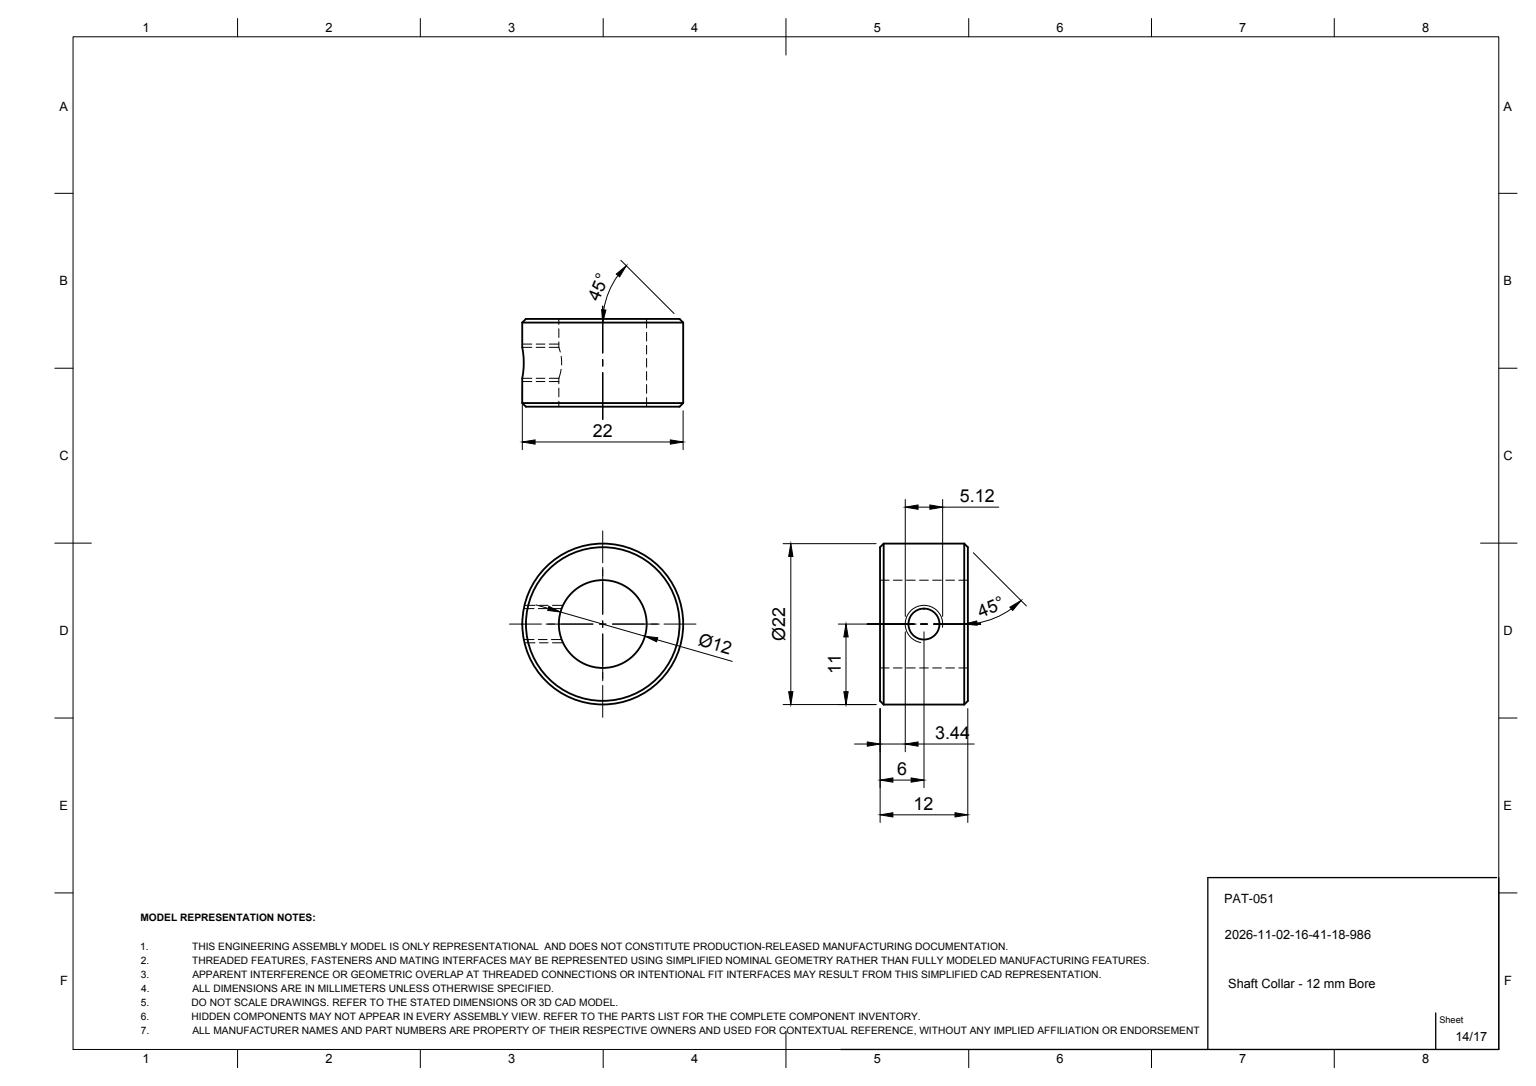
ISO-10303-21;
HEADER;
/* Generated by software containing ST-Developer
 * from STEP Tools, Inc. (www.steptools.com) 
 */

FILE_DESCRIPTION(
/* description */ ('Hand-crank flanged shaft unit'),
/* implementation_level */ '2;1');

FILE_NAME(
/* name */ 'Shaft Collar - 12 mm Bore.step',
/* time_stamp */ '2026-10-27T18:35:45-07:00',
/* author */ (''),
/* organization */ (''),
/* preprocessor_version */ 'ST-DEVELOPER v20.2',
/* originating_system */ 'Autodesk Translation Framework v15.17.0.0',
/* authorisation */ '');

FILE_SCHEMA (('AUTOMOTIVE_DESIGN { 1 0 10303 214 3 1 1 }'));
ENDSEC;

DATA;
#10=MECHANICAL_DESIGN_GEOMETRIC_PRESENTATION_REPRESENTATION('',(#298),#6805);
#24=CONICAL_SURFACE('',#3900,1.075,0.785398163397448);
#25=CONICAL_SURFACE('',#3904,1.075,0.785398163397449);
#235=B_SPLINE_CURVE_WITH_KNOTS('',3,(#6600,#6601,#6602,#6603,#6604,#6605,
#6606,#6607,#6608,#6609,#6610,#6611,#6612,#6613,#6614,#6615,#6616,#6617,
#6618,#6619,#6620,#6621,#6622,#6623,#6624,#6625,#6626,#6627,#6628,#6629,
#6630,#6631,#6632,#6633),.UNSPECIFIED.,.T.,.F.,(4,2,2,2,2,2,2,2,2,2,2,2,
2,2,2,2,4),(0.,0.0805240527913139,0.161048105582628,0.241524630728584,0.322001155874541,
0.402477681020498,0.482954206166455,0.563478258957768,0.644002311749082,
0.724526364540396,0.80505041733171,0.885526942477667,0.966003467623624,
1.04647999276958,1.12695651791554,1.20748057070685,1.28800462349816),
 .UNSPECIFIED.);
#236=B_SPLINE_CURVE_WITH_KNOTS('',3,(#6636,#6637,#6638,#6639,#6640,#6641,
#6642,#6643,#6644,#6645,#6646,#6647,#6648,#6649,#6650,#6651,#6652,#6653,
#6654,#6655,#6656,#6657,#6658,#6659,#6660,#6661,#6662,#6663,#6664,#6665,
#6666,#6667,#6668,#6669),.UNSPECIFIED.,.T.,.F.,(4,2,2,2,2,2,2,2,2,2,2,2,
2,2,2,2,4),(0.,0.0799614062161292,0.159922812432258,0.239880387792505,0.319837963152752,
0.399795538512999,0.479753113873245,0.559714520089374,0.639675926305503,
0.719637332521632,0.799598738737761,0.879556314098008,0.959513889458255,
1.0394714648185,1.11942904017875,1.19939044639488,1.27935185261101),
 .UNSPECIFIED.);
#257=SHAPE_REPRESENTATION_RELATIONSHIP('SRR','None',#6920,#277);
#277=ADVANCED_BREP_SHAPE_REPRESENTATION('',(#318),#6803);
#298=STYLED_ITEM('',(#7091),#318);
#318=MANIFOLD_SOLID_BREP('Body1',#3340);
#405=FACE_BOUND('',#959,.T.);
#406=FACE_BOUND('',#962,.T.);
#407=FACE_BOUND('',#965,.T.);
#408=FACE_BOUND('',#967,.T.);
#504=PLANE('',#3897);
#505=PLANE('',#3906);
#684=FACE_OUTER_BOUND('',#957,.T.);
#685=FACE_OUTER_BOUND('',#958,.T.);
#686=FACE_OUTER_BOUND('',#960,.T.);
#687=FACE_OUTER_BOUND('',#961,.T.);
#688=FACE_OUTER_BOUND('',#963,.T.);
#689=FACE_OUTER_BOUND('',#964,.T.);
#690=FACE_OUTER_BOUND('',#966,.T.);
#957=EDGE_LOOP('',(#2991,#2992,#2993,#2994));
#958=EDGE_LOOP('',(#2995));
#959=EDGE_LOOP('',(#2996));
#960=EDGE_LOOP('',(#2997,#2998,#2999,#3000));
#961=EDGE_LOOP('',(#3001,#3002,#3003,#3004));
#962=EDGE_LOOP('',(#3005));
#963=EDGE_LOOP('',(#3006,#3007,#3008,#3009));
#964=EDGE_LOOP('',(#3010));
#965=EDGE_LOOP('',(#3011));
#966=EDGE_LOOP('',(#3012,#3013,#3014,#3015));
#967=EDGE_LOOP('',(#3016));
#1183=LINE('',#6635,#1411);
#1184=LINE('',#6678,#1412);
#1185=LINE('',#6682,#1413);
#1186=LINE('',#6686,#1414);
#1187=LINE('',#6691,#1415);
#1411=VECTOR('',#4828,0.21);
#1412=VECTOR('',#4839,1.075);
#1413=VECTOR('',#4844,1.1);
#1414=VECTOR('',#4849,1.075);
#1415=VECTOR('',#4856,0.6);
#1559=CIRCLE('',#3898,1.05);
#1560=CIRCLE('',#3899,0.6);
#1561=CIRCLE('',#3901,1.1);
#1562=CIRCLE('',#3903,1.1);
#1563=CIRCLE('',#3905,1.05);
#1564=CIRCLE('',#3907,0.6);
#1819=VERTEX_POINT('',#6599);
#1820=VERTEX_POINT('',#6634);
#1821=VERTEX_POINT('',#6671);
#1822=VERTEX_POINT('',#6673);
#1823=VERTEX_POINT('',#6676);
#1824=VERTEX_POINT('',#6680);
#1825=VERTEX_POINT('',#6684);
#1826=VERTEX_POINT('',#6688);
#2213=EDGE_CURVE('',#1819,#1819,#235,.T.);
#2214=EDGE_CURVE('',#1819,#1820,#1183,.T.);
#2215=EDGE_CURVE('',#1820,#1820,#236,.T.);
#2216=EDGE_CURVE('',#1821,#1821,#1559,.T.);
#2217=EDGE_CURVE('',#1822,#1822,#1560,.T.);
#2218=EDGE_CURVE('',#1823,#1823,#1561,.T.);
#2219=EDGE_CURVE('',#1823,#1821,#1184,.T.);
#2220=EDGE_CURVE('',#1824,#1824,#1562,.T.);
#2221=EDGE_CURVE('',#1824,#1823,#1185,.T.);
#2222=EDGE_CURVE('',#1825,#1825,#1563,.T.);
#2223=EDGE_CURVE('',#1825,#1824,#1186,.T.);
#2224=EDGE_CURVE('',#1826,#1826,#1564,.T.);
#2225=EDGE_CURVE('',#1826,#1822,#1187,.T.);
#2991=ORIENTED_EDGE('',*,*,#2213,.F.);
#2992=ORIENTED_EDGE('',*,*,#2214,.T.);
#2993=ORIENTED_EDGE('',*,*,#2215,.F.);
#2994=ORIENTED_EDGE('',*,*,#2214,.F.);
#2995=ORIENTED_EDGE('',*,*,#2216,.F.);
#2996=ORIENTED_EDGE('',*,*,#2217,.T.);
#2997=ORIENTED_EDGE('',*,*,#2218,.F.);
#2998=ORIENTED_EDGE('',*,*,#2219,.T.);
#2999=ORIENTED_EDGE('',*,*,#2216,.T.);
#3000=ORIENTED_EDGE('',*,*,#2219,.F.);
#3001=ORIENTED_EDGE('',*,*,#2220,.F.);
#3002=ORIENTED_EDGE('',*,*,#2221,.T.);
#3003=ORIENTED_EDGE('',*,*,#2218,.T.);
#3004=ORIENTED_EDGE('',*,*,#2221,.F.);
#3005=ORIENTED_EDGE('',*,*,#2215,.T.);
#3006=ORIENTED_EDGE('',*,*,#2222,.F.);
#3007=ORIENTED_EDGE('',*,*,#2223,.T.);
#3008=ORIENTED_EDGE('',*,*,#2220,.T.);
#3009=ORIENTED_EDGE('',*,*,#2223,.F.);
#3010=ORIENTED_EDGE('',*,*,#2222,.T.);
#3011=ORIENTED_EDGE('',*,*,#2224,.F.);
#3012=ORIENTED_EDGE('',*,*,#2224,.T.);
#3013=ORIENTED_EDGE('',*,*,#2225,.T.);
#3014=ORIENTED_EDGE('',*,*,#2217,.F.);
#3015=ORIENTED_EDGE('',*,*,#2225,.F.);
#3016=ORIENTED_EDGE('',*,*,#2213,.T.);
#3128=CYLINDRICAL_SURFACE('',#3896,0.2117);
#3129=CYLINDRICAL_SURFACE('',#3902,1.1);
#3130=CYLINDRICAL_SURFACE('',#3908,0.6);
#3301=ADVANCED_FACE('',(#684),#3128,.F.);
#3302=ADVANCED_FACE('',(#685,#405),#504,.T.);
#3303=ADVANCED_FACE('',(#686),#24,.T.);
#3304=ADVANCED_FACE('',(#687,#406),#3129,.T.);
#3305=ADVANCED_FACE('',(#688),#25,.T.);
#3306=ADVANCED_FACE('',(#689,#407),#505,.T.);
#3307=ADVANCED_FACE('',(#690,#408),#3130,.F.);
#3340=CLOSED_SHELL('',(#3301,#3302,#3303,#3304,#3305,#3306,#3307));
#3895=AXIS2_PLACEMENT_3D('',#6597,#4824,#4825);
#3896=AXIS2_PLACEMENT_3D('',#6598,#4826,#4827);
#3897=AXIS2_PLACEMENT_3D('',#6670,#4829,#4830);
#3898=AXIS2_PLACEMENT_3D('',#6672,#4831,#4832);
#3899=AXIS2_PLACEMENT_3D('',#6674,#4833,#4834);
#3900=AXIS2_PLACEMENT_3D('',#6675,#4835,#4836);
#3901=AXIS2_PLACEMENT_3D('',#6677,#4837,#4838);
#3902=AXIS2_PLACEMENT_3D('',#6679,#4840,#4841);
#3903=AXIS2_PLACEMENT_3D('',#6681,#4842,#4843);
#3904=AXIS2_PLACEMENT_3D('',#6683,#4845,#4846);
#3905=AXIS2_PLACEMENT_3D('',#6685,#4847,#4848);
#3906=AXIS2_PLACEMENT_3D('',#6687,#4850,#4851);
#3907=AXIS2_PLACEMENT_3D('',#6689,#4852,#4853);
#3908=AXIS2_PLACEMENT_3D('',#6690,#4854,#4855);
#4824=DIRECTION('axis',(0.,0.,1.));
#4825=DIRECTION('refdir',(1.,0.,0.));
#4826=DIRECTION('center_axis',(1.,0.,0.));
#4827=DIRECTION('ref_axis',(0.,0.,-1.));
#4828=DIRECTION('',(1.,0.,0.));
#4829=DIRECTION('center_axis',(0.,1.,0.));
#4830=DIRECTION('ref_axis',(0.,0.,1.));
#4831=DIRECTION('center_axis',(0.,-1.,0.));
#4832=DIRECTION('ref_axis',(1.,0.,0.));
#4833=DIRECTION('center_axis',(0.,-1.,0.));
#4834=DIRECTION('ref_axis',(1.,0.,0.));
#4835=DIRECTION('center_axis',(0.,-1.,0.));
#4836=DIRECTION('ref_axis',(1.,0.,0.));
#4837=DIRECTION('center_axis',(0.,-1.,0.));
#4838=DIRECTION('ref_axis',(1.,0.,0.));
#4839=DIRECTION('',(0.707106781186548,0.707106781186547,8.65956056235493E-17));
#4840=DIRECTION('center_axis',(0.,-1.,0.));
#4841=DIRECTION('ref_axis',(1.,0.,0.));
#4842=DIRECTION('center_axis',(0.,-1.,0.));
#4843=DIRECTION('ref_axis',(1.,0.,0.));
#4844=DIRECTION('',(0.,1.,0.));
#4845=DIRECTION('center_axis',(0.,1.,0.));
#4846=DIRECTION('ref_axis',(1.,0.,0.));
#4847=DIRECTION('center_axis',(0.,-1.,0.));
#4848=DIRECTION('ref_axis',(1.,0.,0.));
#4849=DIRECTION('',(-0.707106781186548,0.707106781186547,-8.65956056235494E-17));
#4850=DIRECTION('center_axis',(0.,-1.,0.));
#4851=DIRECTION('ref_axis',(0.,0.,-1.));
#4852=DIRECTION('center_axis',(0.,-1.,0.));
#4853=DIRECTION('ref_axis',(1.,0.,0.));
#4854=DIRECTION('center_axis',(0.,-1.,0.));
#4855=DIRECTION('ref_axis',(1.,0.,0.));
#4856=DIRECTION('',(0.,1.,0.));
#6597=CARTESIAN_POINT('',(0.,0.,0.));
#6598=CARTESIAN_POINT('Origin',(0.5,0.6,0.));
#6599=CARTESIAN_POINT('',(0.561411711669787,0.6,0.2117));
#6600=CARTESIAN_POINT('Ctrl Pts',(0.561411711669787,0.6,0.2117));
#6601=CARTESIAN_POINT('Ctrl Pts',(0.561411711669787,0.573158649069562,0.2117));
#6602=CARTESIAN_POINT('Ctrl Pts',(0.563539297838208,0.544705001203387,0.206288194517509));
#6603=CARTESIAN_POINT('Ctrl Pts',(0.571006257413022,0.492626080621549,0.184616375754799));
#6604=CARTESIAN_POINT('Ctrl Pts',(0.576215579648966,0.468977868958045,0.168366880112429));
#6605=CARTESIAN_POINT('Ctrl Pts',(0.585834170098139,0.431644140867814,0.131033152022198));
#6606=CARTESIAN_POINT('Ctrl Pts',(0.590898115435695,0.41538619377614,0.107380608633747));
#6607=CARTESIAN_POINT('Ctrl Pts',(0.598025669508798,0.393708029332882,0.0552854099234836));
#6608=CARTESIAN_POINT('Ctrl Pts',(0.6,0.3883,0.0268255083819855));
#6609=CARTESIAN_POINT('Ctrl Pts',(0.6,0.3883,-0.0268255083819856));
#6610=CARTESIAN_POINT('Ctrl Pts',(0.598025669508798,0.393708029332882,-0.0552854099234837));
#6611=CARTESIAN_POINT('Ctrl Pts',(0.590898115435695,0.41538619377614,-0.107380608633747));
#6612=CARTESIAN_POINT('Ctrl Pts',(0.585834170098139,0.431644140867814,-0.131033152022198));
#6613=CARTESIAN_POINT('Ctrl Pts',(0.576215579648966,0.468977868958045,-0.168366880112429));
#6614=CARTESIAN_POINT('Ctrl Pts',(0.571006257413022,0.49262608062155,-0.184616375754799));
#6615=CARTESIAN_POINT('Ctrl Pts',(0.563539297838207,0.544705001203387,-0.206288194517509));
#6616=CARTESIAN_POINT('Ctrl Pts',(0.561411711669787,0.573158649069562,-0.2117));
#6617=CARTESIAN_POINT('Ctrl Pts',(0.561411711669787,0.626841350930438,-0.2117));
#6618=CARTESIAN_POINT('Ctrl Pts',(0.563539297838207,0.655294998796613,-0.206288194517509));
#6619=CARTESIAN_POINT('Ctrl Pts',(0.571006257413022,0.70737391937845,-0.184616375754799));
#6620=CARTESIAN_POINT('Ctrl Pts',(0.576215579648966,0.731022131041955,-0.168366880112429));
#6621=CARTESIAN_POINT('Ctrl Pts',(0.585834170098139,0.768355859132186,-0.131033152022198));
#6622=CARTESIAN_POINT('Ctrl Pts',(0.590898115435695,0.78461380622386,-0.107380608633747));
#6623=CARTESIAN_POINT('Ctrl Pts',(0.598025669508798,0.806291970667118,-0.0552854099234837));
#6624=CARTESIAN_POINT('Ctrl Pts',(0.6,0.8117,-0.0268255083819856));
#6625=CARTESIAN_POINT('Ctrl Pts',(0.6,0.8117,0.0268255083819855));
#6626=CARTESIAN_POINT('Ctrl Pts',(0.598025669508798,0.806291970667118,0.0552854099234837));
#6627=CARTESIAN_POINT('Ctrl Pts',(0.590898115435695,0.78461380622386,0.107380608633747));
#6628=CARTESIAN_POINT('Ctrl Pts',(0.585834170098139,0.768355859132186,0.131033152022198));
#6629=CARTESIAN_POINT('Ctrl Pts',(0.576215579648966,0.731022131041955,0.168366880112429));
#6630=CARTESIAN_POINT('Ctrl Pts',(0.571006257413022,0.70737391937845,0.184616375754799));
#6631=CARTESIAN_POINT('Ctrl Pts',(0.563539297838207,0.655294998796613,0.206288194517509));
#6632=CARTESIAN_POINT('Ctrl Pts',(0.561411711669787,0.626841350930438,0.2117));
#6633=CARTESIAN_POINT('Ctrl Pts',(0.561411711669787,0.6,0.2117));
#6634=CARTESIAN_POINT('',(1.07943647798284,0.6,0.2117));
#6635=CARTESIAN_POINT('',(0.5,0.6,0.2117));
#6636=CARTESIAN_POINT('Ctrl Pts',(1.07943647798284,0.6,0.2117));
#6637=CARTESIAN_POINT('Ctrl Pts',(1.07943647798284,0.626653802072043,0.2117));
#6638=CARTESIAN_POINT('Ctrl Pts',(1.08052600621577,0.655037401084091,0.206359582618511));
#6639=CARTESIAN_POINT('Ctrl Pts',(1.08443252298676,0.707175401021015,0.18473448130117));
#6640=CARTESIAN_POINT('Ctrl Pts',(1.08718996287164,0.730935702749545,0.168453308404839));
#6641=CARTESIAN_POINT('Ctrl Pts',(1.09234340045893,0.768452409692904,0.13093660146148));
#6642=CARTESIAN_POINT('Ctrl Pts',(1.09507838311905,0.784734286816328,0.107175917083711));
#6643=CARTESIAN_POINT('Ctrl Pts',(1.09893326276149,0.806359899102434,0.0550365908820453));
#6644=CARTESIAN_POINT('Ctrl Pts',(1.1,0.8117,0.0266525251200821));
#6645=CARTESIAN_POINT('Ctrl Pts',(1.1,0.8117,-0.0266525251200823));
#6646=CARTESIAN_POINT('Ctrl Pts',(1.09893326276149,0.806359899102434,-0.0550365908820454));
#6647=CARTESIAN_POINT('Ctrl Pts',(1.09507838311905,0.784734286816328,-0.107175917083711));
#6648=CARTESIAN_POINT('Ctrl Pts',(1.09234340045893,0.768452409692904,-0.130936601461481));
#6649=CARTESIAN_POINT('Ctrl Pts',(1.08718996287164,0.730935702749545,-0.16845330840484));
#6650=CARTESIAN_POINT('Ctrl Pts',(1.08443252298676,0.707175401021015,-0.18473448130117));
#6651=CARTESIAN_POINT('Ctrl Pts',(1.08052600621577,0.655037401084091,-0.206359582618511));
#6652=CARTESIAN_POINT('Ctrl Pts',(1.07943647798284,0.626653802072043,-0.2117));
#6653=CARTESIAN_POINT('Ctrl Pts',(1.07943647798284,0.573346197927957,-0.2117));
#6654=CARTESIAN_POINT('Ctrl Pts',(1.08052600621577,0.544962598915909,-0.206359582618511));
#6655=CARTESIAN_POINT('Ctrl Pts',(1.08443252298676,0.492824598978985,-0.18473448130117));
#6656=CARTESIAN_POINT('Ctrl Pts',(1.08718996287164,0.469064297250455,-0.168453308404839));
#6657=CARTESIAN_POINT('Ctrl Pts',(1.09234340045893,0.431547590307096,-0.13093660146148));
#6658=CARTESIAN_POINT('Ctrl Pts',(1.09507838311905,0.415265713183672,-0.107175917083711));
#6659=CARTESIAN_POINT('Ctrl Pts',(1.09893326276149,0.393640100897566,-0.0550365908820454));
#6660=CARTESIAN_POINT('Ctrl Pts',(1.1,0.3883,-0.0266525251200822));
#6661=CARTESIAN_POINT('Ctrl Pts',(1.1,0.3883,0.0266525251200823));
#6662=CARTESIAN_POINT('Ctrl Pts',(1.09893326276149,0.393640100897566,0.0550365908820454));
#6663=CARTESIAN_POINT('Ctrl Pts',(1.09507838311905,0.415265713183672,0.107175917083711));
#6664=CARTESIAN_POINT('Ctrl Pts',(1.09234340045893,0.431547590307096,0.13093660146148));
#6665=CARTESIAN_POINT('Ctrl Pts',(1.08718996287164,0.469064297250455,0.16845330840484));
#6666=CARTESIAN_POINT('Ctrl Pts',(1.08443252298676,0.492824598978985,0.18473448130117));
#6667=CARTESIAN_POINT('Ctrl Pts',(1.08052600621577,0.544962598915909,0.206359582618511));
#6668=CARTESIAN_POINT('Ctrl Pts',(1.07943647798284,0.573346197927957,0.2117));
#6669=CARTESIAN_POINT('Ctrl Pts',(1.07943647798284,0.6,0.2117));
#6670=CARTESIAN_POINT('Origin',(1.05,1.2,0.));
#6671=CARTESIAN_POINT('',(-1.05,1.2,-1.28587913910472E-16));
#6672=CARTESIAN_POINT('Origin',(0.,1.2,0.));
#6673=CARTESIAN_POINT('',(-0.6,1.2,-7.34788079488412E-17));
#6674=CARTESIAN_POINT('Origin',(0.,1.2,0.));
#6675=CARTESIAN_POINT('Origin',(0.,1.175,0.));
#6676=CARTESIAN_POINT('',(-1.1,1.15,-1.34711147906209E-16));
#6677=CARTESIAN_POINT('Origin',(0.,1.15,0.));
#6678=CARTESIAN_POINT('',(-1.075,1.175,-1.3164953090834E-16));
#6679=CARTESIAN_POINT('Origin',(0.,0.6,0.));
#6680=CARTESIAN_POINT('',(-1.1,0.05,-1.34711147906209E-16));
#6681=CARTESIAN_POINT('Origin',(0.,0.05,0.));
#6682=CARTESIAN_POINT('',(-1.1,0.6,-1.34711147906209E-16));
#6683=CARTESIAN_POINT('Origin',(0.,0.025,0.));
#6684=CARTESIAN_POINT('',(-1.05,-4.5102810375397E-17,-1.28587913910472E-16));
#6685=CARTESIAN_POINT('Origin',(0.,0.,0.));
#6686=CARTESIAN_POINT('',(-1.075,0.025,-1.3164953090834E-16));
#6687=CARTESIAN_POINT('Origin',(0.6,0.,0.));
#6688=CARTESIAN_POINT('',(-0.6,0.,-7.34788079488412E-17));
#6689=CARTESIAN_POINT('Origin',(0.,0.,0.));
#6690=CARTESIAN_POINT('Origin',(0.,0.6,0.));
#6691=CARTESIAN_POINT('',(-0.6,0.6,-7.34788079488412E-17));
#6778=UNCERTAINTY_MEASURE_WITH_UNIT(LENGTH_MEASURE(0.001),#6806,
'DISTANCE_ACCURACY_VALUE',
'Maximum model space distance between geometric entities at asserted c
onnectivities');
#6780=UNCERTAINTY_MEASURE_WITH_UNIT(LENGTH_MEASURE(0.001),#6806,
'DISTANCE_ACCURACY_VALUE',
'Maximum model space distance between geometric entities at asserted c
onnectivities');
#6803=(
GEOMETRIC_REPRESENTATION_CONTEXT(3)
GLOBAL_UNCERTAINTY_ASSIGNED_CONTEXT((#6778))
GLOBAL_UNIT_ASSIGNED_CONTEXT((#6806,#6808,#6809))
REPRESENTATION_CONTEXT('','3D')
);
#6805=(
GEOMETRIC_REPRESENTATION_CONTEXT(3)
GLOBAL_UNCERTAINTY_ASSIGNED_CONTEXT((#6780))
GLOBAL_UNIT_ASSIGNED_CONTEXT((#6806,#6808,#6809))
REPRESENTATION_CONTEXT('','3D')
);
#6806=(
LENGTH_UNIT()
NAMED_UNIT(*)
SI_UNIT(.CENTI.,.METRE.)
);
#6808=(
NAMED_UNIT(*)
PLANE_ANGLE_UNIT()
SI_UNIT($,.RADIAN.)
);
#6809=(
NAMED_UNIT(*)
SI_UNIT($,.STERADIAN.)
SOLID_ANGLE_UNIT()
);
#6832=SHAPE_DEFINITION_REPRESENTATION(#6886,#6920);
#6886=PRODUCT_DEFINITION_SHAPE('',$,#6945);
#6920=SHAPE_REPRESENTATION('',(#3895),#6803);
#6922=PRODUCT_DEFINITION_CONTEXT('part definition',#6996,'design');
#6945=PRODUCT_DEFINITION('Shaft Collar - 12 mm Bore',
'Shaft Collar - 12 mm Bore',#6969,#6922);
#6969=PRODUCT_DEFINITION_FORMATION('',$,#7020);
#6996=APPLICATION_CONTEXT(
'Core Data for Automotive Mechanical Design Process');
#6997=PRODUCT_CONTEXT('part definition',#6996,'mechanical');
#7020=PRODUCT('Shaft Collar - 12 mm Bore','Shaft Collar - 12 mm Bore',
'Shaft Collar - 12 mm Bore',(#6997));
#7085=COLOUR_RGB('Grey',0.48,0.52,0.57);
#7086=FILL_AREA_STYLE_COLOUR('',#7085);
#7087=FILL_AREA_STYLE('',(#7086));
#7088=SURFACE_STYLE_FILL_AREA(#7087);
#7089=SURFACE_SIDE_STYLE('',(#7088));
#7090=SURFACE_STYLE_USAGE(.BOTH.,#7089);
#7091=PRESENTATION_STYLE_ASSIGNMENT((#7090));
ENDSEC;
END-ISO-10303-21;
